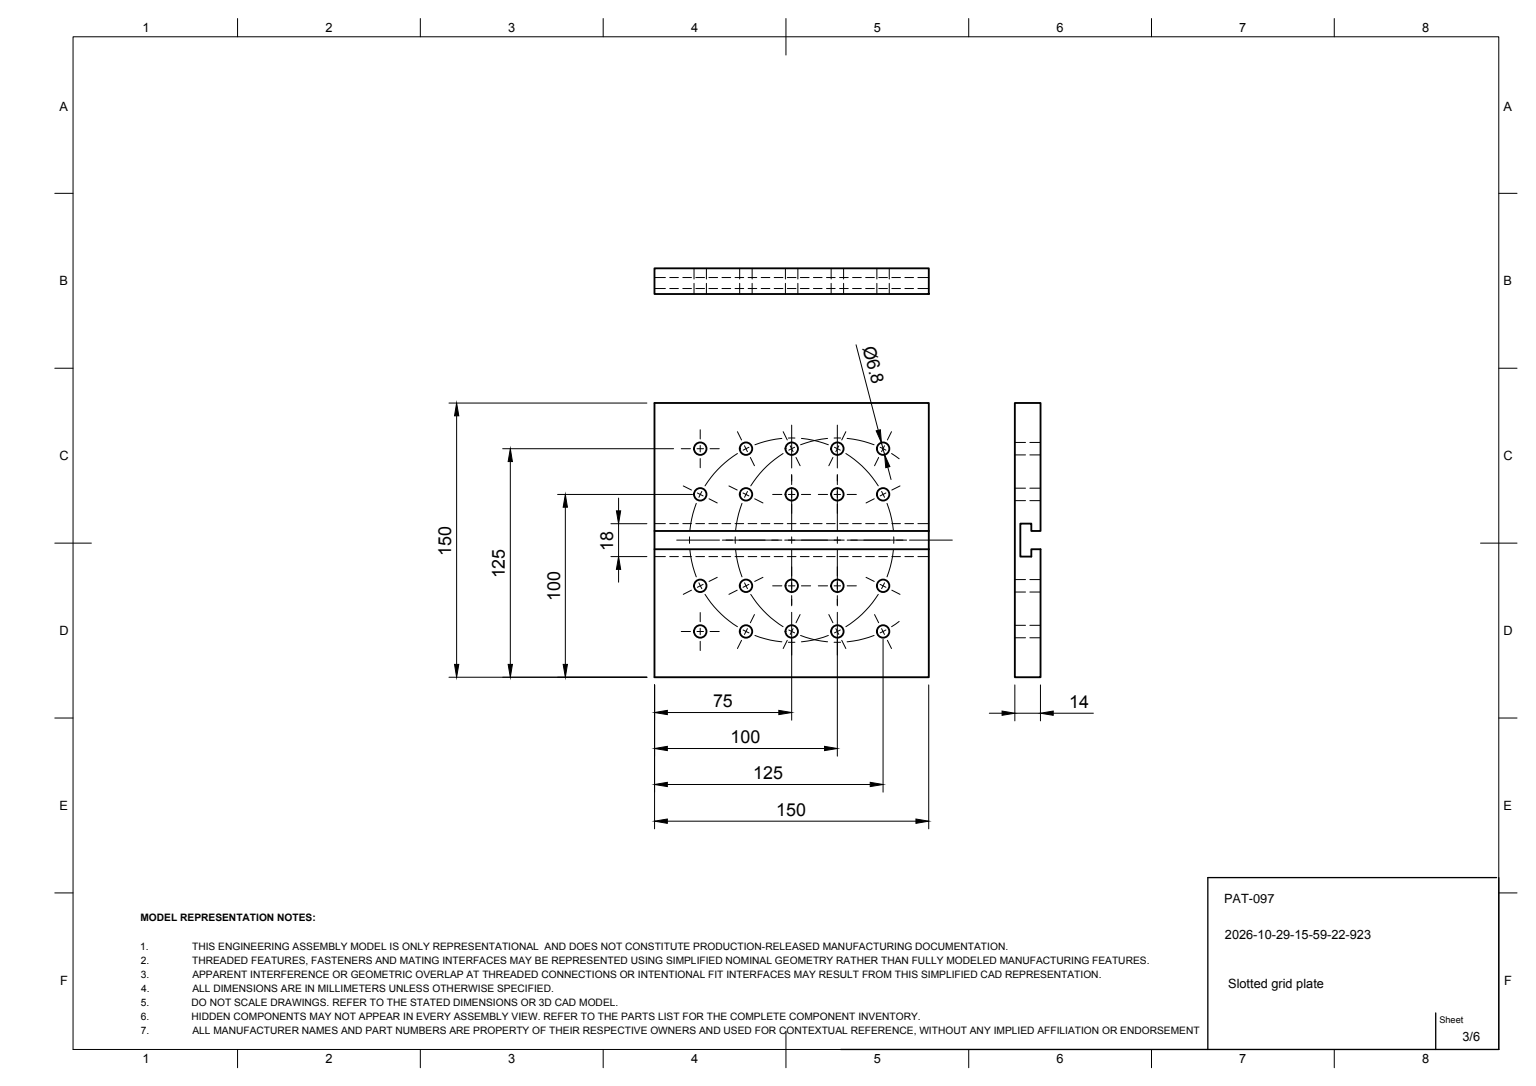
ISO-10303-21;
HEADER;
/* Generated by software containing ST-Developer
 * from STEP Tools, Inc. (www.steptools.com) 
 */

FILE_DESCRIPTION(
/* description */ ('PAT-097'),
/* implementation_level */ '2;1');

FILE_NAME(
/* name */ 'Slotted grid plate.step',
/* time_stamp */ '2026-10-29T15:59:31-07:00',
/* author */ (''),
/* organization */ (''),
/* preprocessor_version */ 'ST-DEVELOPER v20.2',
/* originating_system */ 'Autodesk Translation Framework v15.17.0.0',
/* authorisation */ '');

FILE_SCHEMA (('AUTOMOTIVE_DESIGN { 1 0 10303 214 3 1 1 }'));
ENDSEC;

DATA;
#10=MECHANICAL_DESIGN_GEOMETRIC_PRESENTATION_REPRESENTATION('',(#75),#2768);
#61=SHAPE_REPRESENTATION_RELATIONSHIP('SRR','None',#2799,#68);
#68=ADVANCED_BREP_SHAPE_REPRESENTATION('',(#82),#2761);
#75=STYLED_ITEM('',(#2925),#82);
#82=MANIFOLD_SOLID_BREP('Body1',#1596);
#89=CYLINDRICAL_SURFACE('',#1713,0.34);
#90=CYLINDRICAL_SURFACE('',#1715,0.34);
#91=CYLINDRICAL_SURFACE('',#1717,0.34);
#92=CYLINDRICAL_SURFACE('',#1719,0.34);
#93=CYLINDRICAL_SURFACE('',#1721,0.34);
#94=CYLINDRICAL_SURFACE('',#1723,0.34);
#95=CYLINDRICAL_SURFACE('',#1725,0.34);
#96=CYLINDRICAL_SURFACE('',#1727,0.34);
#97=CYLINDRICAL_SURFACE('',#1729,0.34);
#98=CYLINDRICAL_SURFACE('',#1731,0.34);
#99=CYLINDRICAL_SURFACE('',#1733,0.34);
#100=CYLINDRICAL_SURFACE('',#1735,0.34);
#101=CYLINDRICAL_SURFACE('',#1737,0.34);
#102=CYLINDRICAL_SURFACE('',#1739,0.34);
#103=CYLINDRICAL_SURFACE('',#1741,0.34);
#104=CYLINDRICAL_SURFACE('',#1743,0.34);
#105=CYLINDRICAL_SURFACE('',#1745,0.34);
#106=CYLINDRICAL_SURFACE('',#1747,0.34);
#107=CYLINDRICAL_SURFACE('',#1749,0.34);
#108=CYLINDRICAL_SURFACE('',#1751,0.34);
#116=FACE_BOUND('',#312,.T.);
#117=FACE_BOUND('',#313,.T.);
#118=FACE_BOUND('',#314,.T.);
#119=FACE_BOUND('',#315,.T.);
#120=FACE_BOUND('',#316,.T.);
#121=FACE_BOUND('',#317,.T.);
#122=FACE_BOUND('',#318,.T.);
#123=FACE_BOUND('',#319,.T.);
#124=FACE_BOUND('',#320,.T.);
#125=FACE_BOUND('',#321,.T.);
#126=FACE_BOUND('',#323,.T.);
#127=FACE_BOUND('',#324,.T.);
#128=FACE_BOUND('',#325,.T.);
#129=FACE_BOUND('',#326,.T.);
#130=FACE_BOUND('',#327,.T.);
#131=FACE_BOUND('',#328,.T.);
#132=FACE_BOUND('',#329,.T.);
#133=FACE_BOUND('',#330,.T.);
#134=FACE_BOUND('',#331,.T.);
#135=FACE_BOUND('',#332,.T.);
#136=FACE_BOUND('',#357,.T.);
#137=FACE_BOUND('',#358,.T.);
#138=FACE_BOUND('',#359,.T.);
#139=FACE_BOUND('',#360,.T.);
#140=FACE_BOUND('',#361,.T.);
#141=FACE_BOUND('',#362,.T.);
#142=FACE_BOUND('',#363,.T.);
#143=FACE_BOUND('',#364,.T.);
#144=FACE_BOUND('',#365,.T.);
#145=FACE_BOUND('',#366,.T.);
#146=FACE_BOUND('',#367,.T.);
#147=FACE_BOUND('',#368,.T.);
#148=FACE_BOUND('',#369,.T.);
#149=FACE_BOUND('',#370,.T.);
#150=FACE_BOUND('',#371,.T.);
#151=FACE_BOUND('',#372,.T.);
#152=FACE_BOUND('',#373,.T.);
#153=FACE_BOUND('',#374,.T.);
#154=FACE_BOUND('',#375,.T.);
#155=FACE_BOUND('',#376,.T.);
#164=CIRCLE('',#1692,0.34);
#165=CIRCLE('',#1693,0.34);
#166=CIRCLE('',#1694,0.34);
#167=CIRCLE('',#1695,0.34);
#168=CIRCLE('',#1696,0.34);
#169=CIRCLE('',#1697,0.34);
#170=CIRCLE('',#1698,0.34);
#171=CIRCLE('',#1699,0.34);
#172=CIRCLE('',#1700,0.34);
#173=CIRCLE('',#1701,0.34);
#174=CIRCLE('',#1703,0.34);
#175=CIRCLE('',#1704,0.34);
#176=CIRCLE('',#1705,0.34);
#177=CIRCLE('',#1706,0.34);
#178=CIRCLE('',#1707,0.34);
#179=CIRCLE('',#1708,0.34);
#180=CIRCLE('',#1709,0.34);
#181=CIRCLE('',#1710,0.34);
#182=CIRCLE('',#1711,0.34);
#183=CIRCLE('',#1712,0.34);
#184=CIRCLE('',#1714,0.34);
#185=CIRCLE('',#1716,0.34);
#186=CIRCLE('',#1718,0.34);
#187=CIRCLE('',#1720,0.34);
#188=CIRCLE('',#1722,0.34);
#189=CIRCLE('',#1724,0.34);
#190=CIRCLE('',#1726,0.34);
#191=CIRCLE('',#1728,0.34);
#192=CIRCLE('',#1730,0.34);
#193=CIRCLE('',#1732,0.34);
#194=CIRCLE('',#1734,0.34);
#195=CIRCLE('',#1736,0.34);
#196=CIRCLE('',#1738,0.34);
#197=CIRCLE('',#1740,0.34);
#198=CIRCLE('',#1742,0.34);
#199=CIRCLE('',#1744,0.34);
#200=CIRCLE('',#1746,0.34);
#201=CIRCLE('',#1748,0.34);
#202=CIRCLE('',#1750,0.34);
#203=CIRCLE('',#1752,0.34);
#220=FACE_OUTER_BOUND('',#303,.T.);
#221=FACE_OUTER_BOUND('',#304,.T.);
#222=FACE_OUTER_BOUND('',#305,.T.);
#223=FACE_OUTER_BOUND('',#306,.T.);
#224=FACE_OUTER_BOUND('',#307,.T.);
#225=FACE_OUTER_BOUND('',#308,.T.);
#226=FACE_OUTER_BOUND('',#309,.T.);
#227=FACE_OUTER_BOUND('',#310,.T.);
#228=FACE_OUTER_BOUND('',#311,.T.);
#229=FACE_OUTER_BOUND('',#322,.T.);
#230=FACE_OUTER_BOUND('',#333,.T.);
#231=FACE_OUTER_BOUND('',#334,.T.);
#232=FACE_OUTER_BOUND('',#335,.T.);
#233=FACE_OUTER_BOUND('',#336,.T.);
#234=FACE_OUTER_BOUND('',#337,.T.);
#235=FACE_OUTER_BOUND('',#338,.T.);
#236=FACE_OUTER_BOUND('',#339,.T.);
#237=FACE_OUTER_BOUND('',#340,.T.);
#238=FACE_OUTER_BOUND('',#341,.T.);
#239=FACE_OUTER_BOUND('',#342,.T.);
#240=FACE_OUTER_BOUND('',#343,.T.);
#241=FACE_OUTER_BOUND('',#344,.T.);
#242=FACE_OUTER_BOUND('',#345,.T.);
#243=FACE_OUTER_BOUND('',#346,.T.);
#244=FACE_OUTER_BOUND('',#347,.T.);
#245=FACE_OUTER_BOUND('',#348,.T.);
#246=FACE_OUTER_BOUND('',#349,.T.);
#247=FACE_OUTER_BOUND('',#350,.T.);
#248=FACE_OUTER_BOUND('',#351,.T.);
#249=FACE_OUTER_BOUND('',#352,.T.);
#250=FACE_OUTER_BOUND('',#353,.T.);
#251=FACE_OUTER_BOUND('',#354,.T.);
#252=FACE_OUTER_BOUND('',#355,.T.);
#253=FACE_OUTER_BOUND('',#356,.T.);
#303=EDGE_LOOP('',(#1049,#1050,#1051,#1052));
#304=EDGE_LOOP('',(#1053,#1054,#1055,#1056));
#305=EDGE_LOOP('',(#1057,#1058,#1059,#1060));
#306=EDGE_LOOP('',(#1061,#1062,#1063,#1064));
#307=EDGE_LOOP('',(#1065,#1066,#1067,#1068));
#308=EDGE_LOOP('',(#1069,#1070,#1071,#1072));
#309=EDGE_LOOP('',(#1073,#1074,#1075,#1076));
#310=EDGE_LOOP('',(#1077,#1078,#1079,#1080,#1081,#1082,#1083,#1084,#1085,
#1086,#1087,#1088));
#311=EDGE_LOOP('',(#1089,#1090,#1091,#1092));
#312=EDGE_LOOP('',(#1093));
#313=EDGE_LOOP('',(#1094));
#314=EDGE_LOOP('',(#1095));
#315=EDGE_LOOP('',(#1096));
#316=EDGE_LOOP('',(#1097));
#317=EDGE_LOOP('',(#1098));
#318=EDGE_LOOP('',(#1099));
#319=EDGE_LOOP('',(#1100));
#320=EDGE_LOOP('',(#1101));
#321=EDGE_LOOP('',(#1102));
#322=EDGE_LOOP('',(#1103,#1104,#1105,#1106));
#323=EDGE_LOOP('',(#1107));
#324=EDGE_LOOP('',(#1108));
#325=EDGE_LOOP('',(#1109));
#326=EDGE_LOOP('',(#1110));
#327=EDGE_LOOP('',(#1111));
#328=EDGE_LOOP('',(#1112));
#329=EDGE_LOOP('',(#1113));
#330=EDGE_LOOP('',(#1114));
#331=EDGE_LOOP('',(#1115));
#332=EDGE_LOOP('',(#1116));
#333=EDGE_LOOP('',(#1117,#1118,#1119,#1120));
#334=EDGE_LOOP('',(#1121,#1122,#1123,#1124));
#335=EDGE_LOOP('',(#1125,#1126,#1127,#1128));
#336=EDGE_LOOP('',(#1129,#1130,#1131,#1132));
#337=EDGE_LOOP('',(#1133,#1134,#1135,#1136));
#338=EDGE_LOOP('',(#1137,#1138,#1139,#1140));
#339=EDGE_LOOP('',(#1141,#1142,#1143,#1144));
#340=EDGE_LOOP('',(#1145,#1146,#1147,#1148));
#341=EDGE_LOOP('',(#1149,#1150,#1151,#1152));
#342=EDGE_LOOP('',(#1153,#1154,#1155,#1156));
#343=EDGE_LOOP('',(#1157,#1158,#1159,#1160));
#344=EDGE_LOOP('',(#1161,#1162,#1163,#1164));
#345=EDGE_LOOP('',(#1165,#1166,#1167,#1168));
#346=EDGE_LOOP('',(#1169,#1170,#1171,#1172));
#347=EDGE_LOOP('',(#1173,#1174,#1175,#1176));
#348=EDGE_LOOP('',(#1177,#1178,#1179,#1180));
#349=EDGE_LOOP('',(#1181,#1182,#1183,#1184));
#350=EDGE_LOOP('',(#1185,#1186,#1187,#1188));
#351=EDGE_LOOP('',(#1189,#1190,#1191,#1192));
#352=EDGE_LOOP('',(#1193,#1194,#1195,#1196));
#353=EDGE_LOOP('',(#1197,#1198,#1199,#1200));
#354=EDGE_LOOP('',(#1201,#1202,#1203,#1204,#1205,#1206,#1207,#1208,#1209,
#1210,#1211,#1212));
#355=EDGE_LOOP('',(#1213,#1214,#1215,#1216));
#356=EDGE_LOOP('',(#1217,#1218,#1219,#1220));
#357=EDGE_LOOP('',(#1221));
#358=EDGE_LOOP('',(#1222));
#359=EDGE_LOOP('',(#1223));
#360=EDGE_LOOP('',(#1224));
#361=EDGE_LOOP('',(#1225));
#362=EDGE_LOOP('',(#1226));
#363=EDGE_LOOP('',(#1227));
#364=EDGE_LOOP('',(#1228));
#365=EDGE_LOOP('',(#1229));
#366=EDGE_LOOP('',(#1230));
#367=EDGE_LOOP('',(#1231));
#368=EDGE_LOOP('',(#1232));
#369=EDGE_LOOP('',(#1233));
#370=EDGE_LOOP('',(#1234));
#371=EDGE_LOOP('',(#1235));
#372=EDGE_LOOP('',(#1236));
#373=EDGE_LOOP('',(#1237));
#374=EDGE_LOOP('',(#1238));
#375=EDGE_LOOP('',(#1239));
#376=EDGE_LOOP('',(#1240));
#434=LINE('',#2291,#571);
#435=LINE('',#2293,#572);
#436=LINE('',#2295,#573);
#437=LINE('',#2296,#574);
#438=LINE('',#2299,#575);
#439=LINE('',#2301,#576);
#440=LINE('',#2302,#577);
#441=LINE('',#2306,#578);
#442=LINE('',#2308,#579);
#443=LINE('',#2310,#580);
#444=LINE('',#2311,#581);
#445=LINE('',#2314,#582);
#446=LINE('',#2316,#583);
#447=LINE('',#2317,#584);
#448=LINE('',#2320,#585);
#449=LINE('',#2322,#586);
#450=LINE('',#2323,#587);
#451=LINE('',#2326,#588);
#452=LINE('',#2328,#589);
#453=LINE('',#2329,#590);
#454=LINE('',#2331,#591);
#455=LINE('',#2332,#592);
#456=LINE('',#2335,#593);
#457=LINE('',#2337,#594);
#458=LINE('',#2339,#595);
#459=LINE('',#2341,#596);
#460=LINE('',#2342,#597);
#461=LINE('',#2345,#598);
#462=LINE('',#2346,#599);
#463=LINE('',#2369,#600);
#464=LINE('',#2370,#601);
#465=LINE('',#2394,#602);
#466=LINE('',#2398,#603);
#467=LINE('',#2402,#604);
#468=LINE('',#2406,#605);
#469=LINE('',#2410,#606);
#470=LINE('',#2414,#607);
#471=LINE('',#2418,#608);
#472=LINE('',#2422,#609);
#473=LINE('',#2426,#610);
#474=LINE('',#2430,#611);
#475=LINE('',#2434,#612);
#476=LINE('',#2438,#613);
#477=LINE('',#2442,#614);
#478=LINE('',#2446,#615);
#479=LINE('',#2450,#616);
#480=LINE('',#2454,#617);
#481=LINE('',#2458,#618);
#482=LINE('',#2462,#619);
#483=LINE('',#2466,#620);
#484=LINE('',#2470,#621);
#485=LINE('',#2473,#622);
#486=LINE('',#2474,#623);
#487=LINE('',#2477,#624);
#488=LINE('',#2478,#625);
#489=LINE('',#2480,#626);
#571=VECTOR('',#1843,1.);
#572=VECTOR('',#1844,1.);
#573=VECTOR('',#1845,1.);
#574=VECTOR('',#1846,1.);
#575=VECTOR('',#1849,1.);
#576=VECTOR('',#1850,1.);
#577=VECTOR('',#1851,1.);
#578=VECTOR('',#1854,1.);
#579=VECTOR('',#1855,1.);
#580=VECTOR('',#1856,1.);
#581=VECTOR('',#1857,1.);
#582=VECTOR('',#1860,1.);
#583=VECTOR('',#1861,1.);
#584=VECTOR('',#1862,1.);
#585=VECTOR('',#1865,1.);
#586=VECTOR('',#1866,1.);
#587=VECTOR('',#1867,1.);
#588=VECTOR('',#1870,1.);
#589=VECTOR('',#1871,1.);
#590=VECTOR('',#1872,1.);
#591=VECTOR('',#1875,1.);
#592=VECTOR('',#1876,1.);
#593=VECTOR('',#1879,1.);
#594=VECTOR('',#1880,1.);
#595=VECTOR('',#1881,1.);
#596=VECTOR('',#1882,1.);
#597=VECTOR('',#1883,1.);
#598=VECTOR('',#1886,1.);
#599=VECTOR('',#1887,1.);
#600=VECTOR('',#1910,1.);
#601=VECTOR('',#1911,1.);
#602=VECTOR('',#1936,0.34);
#603=VECTOR('',#1941,0.34);
#604=VECTOR('',#1946,0.34);
#605=VECTOR('',#1951,0.34);
#606=VECTOR('',#1956,0.34);
#607=VECTOR('',#1961,0.34);
#608=VECTOR('',#1966,0.34);
#609=VECTOR('',#1971,0.34);
#610=VECTOR('',#1976,0.34);
#611=VECTOR('',#1981,0.34);
#612=VECTOR('',#1986,0.34);
#613=VECTOR('',#1991,0.34);
#614=VECTOR('',#1996,0.34);
#615=VECTOR('',#2001,0.34);
#616=VECTOR('',#2006,0.34);
#617=VECTOR('',#2011,0.34);
#618=VECTOR('',#2016,0.34);
#619=VECTOR('',#2021,0.34);
#620=VECTOR('',#2026,0.34);
#621=VECTOR('',#2031,0.34);
#622=VECTOR('',#2034,1.);
#623=VECTOR('',#2035,1.);
#624=VECTOR('',#2038,1.);
#625=VECTOR('',#2039,1.);
#626=VECTOR('',#2042,1.);
#708=VERTEX_POINT('',#2289);
#709=VERTEX_POINT('',#2290);
#710=VERTEX_POINT('',#2292);
#711=VERTEX_POINT('',#2294);
#712=VERTEX_POINT('',#2298);
#713=VERTEX_POINT('',#2300);
#714=VERTEX_POINT('',#2304);
#715=VERTEX_POINT('',#2305);
#716=VERTEX_POINT('',#2307);
#717=VERTEX_POINT('',#2309);
#718=VERTEX_POINT('',#2313);
#719=VERTEX_POINT('',#2315);
#720=VERTEX_POINT('',#2319);
#721=VERTEX_POINT('',#2321);
#722=VERTEX_POINT('',#2325);
#723=VERTEX_POINT('',#2327);
#724=VERTEX_POINT('',#2334);
#725=VERTEX_POINT('',#2336);
#726=VERTEX_POINT('',#2338);
#727=VERTEX_POINT('',#2340);
#728=VERTEX_POINT('',#2344);
#729=VERTEX_POINT('',#2347);
#730=VERTEX_POINT('',#2349);
#731=VERTEX_POINT('',#2351);
#732=VERTEX_POINT('',#2353);
#733=VERTEX_POINT('',#2355);
#734=VERTEX_POINT('',#2357);
#735=VERTEX_POINT('',#2359);
#736=VERTEX_POINT('',#2361);
#737=VERTEX_POINT('',#2363);
#738=VERTEX_POINT('',#2365);
#739=VERTEX_POINT('',#2368);
#740=VERTEX_POINT('',#2371);
#741=VERTEX_POINT('',#2373);
#742=VERTEX_POINT('',#2375);
#743=VERTEX_POINT('',#2377);
#744=VERTEX_POINT('',#2379);
#745=VERTEX_POINT('',#2381);
#746=VERTEX_POINT('',#2383);
#747=VERTEX_POINT('',#2385);
#748=VERTEX_POINT('',#2387);
#749=VERTEX_POINT('',#2389);
#750=VERTEX_POINT('',#2392);
#751=VERTEX_POINT('',#2396);
#752=VERTEX_POINT('',#2400);
#753=VERTEX_POINT('',#2404);
#754=VERTEX_POINT('',#2408);
#755=VERTEX_POINT('',#2412);
#756=VERTEX_POINT('',#2416);
#757=VERTEX_POINT('',#2420);
#758=VERTEX_POINT('',#2424);
#759=VERTEX_POINT('',#2428);
#760=VERTEX_POINT('',#2432);
#761=VERTEX_POINT('',#2436);
#762=VERTEX_POINT('',#2440);
#763=VERTEX_POINT('',#2444);
#764=VERTEX_POINT('',#2448);
#765=VERTEX_POINT('',#2452);
#766=VERTEX_POINT('',#2456);
#767=VERTEX_POINT('',#2460);
#768=VERTEX_POINT('',#2464);
#769=VERTEX_POINT('',#2468);
#770=VERTEX_POINT('',#2472);
#771=VERTEX_POINT('',#2476);
#844=EDGE_CURVE('',#708,#709,#434,.T.);
#845=EDGE_CURVE('',#710,#708,#435,.T.);
#846=EDGE_CURVE('',#711,#710,#436,.T.);
#847=EDGE_CURVE('',#709,#711,#437,.T.);
#848=EDGE_CURVE('',#712,#708,#438,.T.);
#849=EDGE_CURVE('',#713,#712,#439,.T.);
#850=EDGE_CURVE('',#710,#713,#440,.T.);
#851=EDGE_CURVE('',#714,#715,#441,.T.);
#852=EDGE_CURVE('',#716,#714,#442,.T.);
#853=EDGE_CURVE('',#717,#716,#443,.T.);
#854=EDGE_CURVE('',#717,#715,#444,.T.);
#855=EDGE_CURVE('',#715,#718,#445,.T.);
#856=EDGE_CURVE('',#719,#717,#446,.T.);
#857=EDGE_CURVE('',#719,#718,#447,.T.);
#858=EDGE_CURVE('',#718,#720,#448,.T.);
#859=EDGE_CURVE('',#721,#719,#449,.T.);
#860=EDGE_CURVE('',#721,#720,#450,.T.);
#861=EDGE_CURVE('',#720,#722,#451,.T.);
#862=EDGE_CURVE('',#723,#721,#452,.T.);
#863=EDGE_CURVE('',#723,#722,#453,.T.);
#864=EDGE_CURVE('',#722,#712,#454,.T.);
#865=EDGE_CURVE('',#713,#723,#455,.T.);
#866=EDGE_CURVE('',#724,#716,#456,.T.);
#867=EDGE_CURVE('',#725,#724,#457,.T.);
#868=EDGE_CURVE('',#725,#726,#458,.T.);
#869=EDGE_CURVE('',#726,#727,#459,.T.);
#870=EDGE_CURVE('',#711,#727,#460,.T.);
#871=EDGE_CURVE('',#714,#728,#461,.T.);
#872=EDGE_CURVE('',#728,#724,#462,.T.);
#873=EDGE_CURVE('',#729,#729,#164,.T.);
#874=EDGE_CURVE('',#730,#730,#165,.T.);
#875=EDGE_CURVE('',#731,#731,#166,.T.);
#876=EDGE_CURVE('',#732,#732,#167,.T.);
#877=EDGE_CURVE('',#733,#733,#168,.T.);
#878=EDGE_CURVE('',#734,#734,#169,.T.);
#879=EDGE_CURVE('',#735,#735,#170,.T.);
#880=EDGE_CURVE('',#736,#736,#171,.T.);
#881=EDGE_CURVE('',#737,#737,#172,.T.);
#882=EDGE_CURVE('',#738,#738,#173,.T.);
#883=EDGE_CURVE('',#727,#739,#463,.T.);
#884=EDGE_CURVE('',#739,#709,#464,.T.);
#885=EDGE_CURVE('',#740,#740,#174,.T.);
#886=EDGE_CURVE('',#741,#741,#175,.T.);
#887=EDGE_CURVE('',#742,#742,#176,.T.);
#888=EDGE_CURVE('',#743,#743,#177,.T.);
#889=EDGE_CURVE('',#744,#744,#178,.T.);
#890=EDGE_CURVE('',#745,#745,#179,.T.);
#891=EDGE_CURVE('',#746,#746,#180,.T.);
#892=EDGE_CURVE('',#747,#747,#181,.T.);
#893=EDGE_CURVE('',#748,#748,#182,.T.);
#894=EDGE_CURVE('',#749,#749,#183,.T.);
#895=EDGE_CURVE('',#750,#750,#184,.T.);
#896=EDGE_CURVE('',#750,#729,#465,.T.);
#897=EDGE_CURVE('',#751,#751,#185,.T.);
#898=EDGE_CURVE('',#751,#740,#466,.T.);
#899=EDGE_CURVE('',#752,#752,#186,.T.);
#900=EDGE_CURVE('',#752,#730,#467,.T.);
#901=EDGE_CURVE('',#753,#753,#187,.T.);
#902=EDGE_CURVE('',#753,#741,#468,.T.);
#903=EDGE_CURVE('',#754,#754,#188,.T.);
#904=EDGE_CURVE('',#754,#731,#469,.T.);
#905=EDGE_CURVE('',#755,#755,#189,.T.);
#906=EDGE_CURVE('',#755,#742,#470,.T.);
#907=EDGE_CURVE('',#756,#756,#190,.T.);
#908=EDGE_CURVE('',#756,#732,#471,.T.);
#909=EDGE_CURVE('',#757,#757,#191,.T.);
#910=EDGE_CURVE('',#757,#743,#472,.T.);
#911=EDGE_CURVE('',#758,#758,#192,.T.);
#912=EDGE_CURVE('',#758,#733,#473,.T.);
#913=EDGE_CURVE('',#759,#759,#193,.T.);
#914=EDGE_CURVE('',#759,#744,#474,.T.);
#915=EDGE_CURVE('',#760,#760,#194,.T.);
#916=EDGE_CURVE('',#760,#734,#475,.T.);
#917=EDGE_CURVE('',#761,#761,#195,.T.);
#918=EDGE_CURVE('',#761,#745,#476,.T.);
#919=EDGE_CURVE('',#762,#762,#196,.T.);
#920=EDGE_CURVE('',#762,#735,#477,.T.);
#921=EDGE_CURVE('',#763,#763,#197,.T.);
#922=EDGE_CURVE('',#763,#746,#478,.T.);
#923=EDGE_CURVE('',#764,#764,#198,.T.);
#924=EDGE_CURVE('',#764,#747,#479,.T.);
#925=EDGE_CURVE('',#765,#765,#199,.T.);
#926=EDGE_CURVE('',#765,#736,#480,.T.);
#927=EDGE_CURVE('',#766,#766,#200,.T.);
#928=EDGE_CURVE('',#766,#748,#481,.T.);
#929=EDGE_CURVE('',#767,#767,#201,.T.);
#930=EDGE_CURVE('',#767,#737,#482,.T.);
#931=EDGE_CURVE('',#768,#768,#202,.T.);
#932=EDGE_CURVE('',#768,#749,#483,.T.);
#933=EDGE_CURVE('',#769,#769,#203,.T.);
#934=EDGE_CURVE('',#769,#738,#484,.T.);
#935=EDGE_CURVE('',#770,#725,#485,.T.);
#936=EDGE_CURVE('',#770,#728,#486,.T.);
#937=EDGE_CURVE('',#771,#739,#487,.T.);
#938=EDGE_CURVE('',#771,#770,#488,.T.);
#939=EDGE_CURVE('',#726,#771,#489,.T.);
#1049=ORIENTED_EDGE('',*,*,#844,.F.);
#1050=ORIENTED_EDGE('',*,*,#845,.F.);
#1051=ORIENTED_EDGE('',*,*,#846,.F.);
#1052=ORIENTED_EDGE('',*,*,#847,.F.);
#1053=ORIENTED_EDGE('',*,*,#848,.F.);
#1054=ORIENTED_EDGE('',*,*,#849,.F.);
#1055=ORIENTED_EDGE('',*,*,#850,.F.);
#1056=ORIENTED_EDGE('',*,*,#845,.T.);
#1057=ORIENTED_EDGE('',*,*,#851,.F.);
#1058=ORIENTED_EDGE('',*,*,#852,.F.);
#1059=ORIENTED_EDGE('',*,*,#853,.F.);
#1060=ORIENTED_EDGE('',*,*,#854,.T.);
#1061=ORIENTED_EDGE('',*,*,#855,.F.);
#1062=ORIENTED_EDGE('',*,*,#854,.F.);
#1063=ORIENTED_EDGE('',*,*,#856,.F.);
#1064=ORIENTED_EDGE('',*,*,#857,.T.);
#1065=ORIENTED_EDGE('',*,*,#858,.F.);
#1066=ORIENTED_EDGE('',*,*,#857,.F.);
#1067=ORIENTED_EDGE('',*,*,#859,.F.);
#1068=ORIENTED_EDGE('',*,*,#860,.T.);
#1069=ORIENTED_EDGE('',*,*,#861,.F.);
#1070=ORIENTED_EDGE('',*,*,#860,.F.);
#1071=ORIENTED_EDGE('',*,*,#862,.F.);
#1072=ORIENTED_EDGE('',*,*,#863,.T.);
#1073=ORIENTED_EDGE('',*,*,#864,.F.);
#1074=ORIENTED_EDGE('',*,*,#863,.F.);
#1075=ORIENTED_EDGE('',*,*,#865,.F.);
#1076=ORIENTED_EDGE('',*,*,#849,.T.);
#1077=ORIENTED_EDGE('',*,*,#846,.T.);
#1078=ORIENTED_EDGE('',*,*,#850,.T.);
#1079=ORIENTED_EDGE('',*,*,#865,.T.);
#1080=ORIENTED_EDGE('',*,*,#862,.T.);
#1081=ORIENTED_EDGE('',*,*,#859,.T.);
#1082=ORIENTED_EDGE('',*,*,#856,.T.);
#1083=ORIENTED_EDGE('',*,*,#853,.T.);
#1084=ORIENTED_EDGE('',*,*,#866,.F.);
#1085=ORIENTED_EDGE('',*,*,#867,.F.);
#1086=ORIENTED_EDGE('',*,*,#868,.T.);
#1087=ORIENTED_EDGE('',*,*,#869,.T.);
#1088=ORIENTED_EDGE('',*,*,#870,.F.);
#1089=ORIENTED_EDGE('',*,*,#852,.T.);
#1090=ORIENTED_EDGE('',*,*,#871,.T.);
#1091=ORIENTED_EDGE('',*,*,#872,.T.);
#1092=ORIENTED_EDGE('',*,*,#866,.T.);
#1093=ORIENTED_EDGE('',*,*,#873,.T.);
#1094=ORIENTED_EDGE('',*,*,#874,.T.);
#1095=ORIENTED_EDGE('',*,*,#875,.T.);
#1096=ORIENTED_EDGE('',*,*,#876,.T.);
#1097=ORIENTED_EDGE('',*,*,#877,.T.);
#1098=ORIENTED_EDGE('',*,*,#878,.T.);
#1099=ORIENTED_EDGE('',*,*,#879,.T.);
#1100=ORIENTED_EDGE('',*,*,#880,.T.);
#1101=ORIENTED_EDGE('',*,*,#881,.T.);
#1102=ORIENTED_EDGE('',*,*,#882,.T.);
#1103=ORIENTED_EDGE('',*,*,#847,.T.);
#1104=ORIENTED_EDGE('',*,*,#870,.T.);
#1105=ORIENTED_EDGE('',*,*,#883,.T.);
#1106=ORIENTED_EDGE('',*,*,#884,.T.);
#1107=ORIENTED_EDGE('',*,*,#885,.T.);
#1108=ORIENTED_EDGE('',*,*,#886,.T.);
#1109=ORIENTED_EDGE('',*,*,#887,.T.);
#1110=ORIENTED_EDGE('',*,*,#888,.T.);
#1111=ORIENTED_EDGE('',*,*,#889,.T.);
#1112=ORIENTED_EDGE('',*,*,#890,.T.);
#1113=ORIENTED_EDGE('',*,*,#891,.T.);
#1114=ORIENTED_EDGE('',*,*,#892,.T.);
#1115=ORIENTED_EDGE('',*,*,#893,.T.);
#1116=ORIENTED_EDGE('',*,*,#894,.T.);
#1117=ORIENTED_EDGE('',*,*,#895,.F.);
#1118=ORIENTED_EDGE('',*,*,#896,.T.);
#1119=ORIENTED_EDGE('',*,*,#873,.F.);
#1120=ORIENTED_EDGE('',*,*,#896,.F.);
#1121=ORIENTED_EDGE('',*,*,#897,.F.);
#1122=ORIENTED_EDGE('',*,*,#898,.T.);
#1123=ORIENTED_EDGE('',*,*,#885,.F.);
#1124=ORIENTED_EDGE('',*,*,#898,.F.);
#1125=ORIENTED_EDGE('',*,*,#899,.F.);
#1126=ORIENTED_EDGE('',*,*,#900,.T.);
#1127=ORIENTED_EDGE('',*,*,#874,.F.);
#1128=ORIENTED_EDGE('',*,*,#900,.F.);
#1129=ORIENTED_EDGE('',*,*,#901,.F.);
#1130=ORIENTED_EDGE('',*,*,#902,.T.);
#1131=ORIENTED_EDGE('',*,*,#886,.F.);
#1132=ORIENTED_EDGE('',*,*,#902,.F.);
#1133=ORIENTED_EDGE('',*,*,#903,.F.);
#1134=ORIENTED_EDGE('',*,*,#904,.T.);
#1135=ORIENTED_EDGE('',*,*,#875,.F.);
#1136=ORIENTED_EDGE('',*,*,#904,.F.);
#1137=ORIENTED_EDGE('',*,*,#905,.F.);
#1138=ORIENTED_EDGE('',*,*,#906,.T.);
#1139=ORIENTED_EDGE('',*,*,#887,.F.);
#1140=ORIENTED_EDGE('',*,*,#906,.F.);
#1141=ORIENTED_EDGE('',*,*,#907,.F.);
#1142=ORIENTED_EDGE('',*,*,#908,.T.);
#1143=ORIENTED_EDGE('',*,*,#876,.F.);
#1144=ORIENTED_EDGE('',*,*,#908,.F.);
#1145=ORIENTED_EDGE('',*,*,#909,.F.);
#1146=ORIENTED_EDGE('',*,*,#910,.T.);
#1147=ORIENTED_EDGE('',*,*,#888,.F.);
#1148=ORIENTED_EDGE('',*,*,#910,.F.);
#1149=ORIENTED_EDGE('',*,*,#911,.F.);
#1150=ORIENTED_EDGE('',*,*,#912,.T.);
#1151=ORIENTED_EDGE('',*,*,#877,.F.);
#1152=ORIENTED_EDGE('',*,*,#912,.F.);
#1153=ORIENTED_EDGE('',*,*,#913,.F.);
#1154=ORIENTED_EDGE('',*,*,#914,.T.);
#1155=ORIENTED_EDGE('',*,*,#889,.F.);
#1156=ORIENTED_EDGE('',*,*,#914,.F.);
#1157=ORIENTED_EDGE('',*,*,#915,.F.);
#1158=ORIENTED_EDGE('',*,*,#916,.T.);
#1159=ORIENTED_EDGE('',*,*,#878,.F.);
#1160=ORIENTED_EDGE('',*,*,#916,.F.);
#1161=ORIENTED_EDGE('',*,*,#917,.F.);
#1162=ORIENTED_EDGE('',*,*,#918,.T.);
#1163=ORIENTED_EDGE('',*,*,#890,.F.);
#1164=ORIENTED_EDGE('',*,*,#918,.F.);
#1165=ORIENTED_EDGE('',*,*,#919,.F.);
#1166=ORIENTED_EDGE('',*,*,#920,.T.);
#1167=ORIENTED_EDGE('',*,*,#879,.F.);
#1168=ORIENTED_EDGE('',*,*,#920,.F.);
#1169=ORIENTED_EDGE('',*,*,#921,.F.);
#1170=ORIENTED_EDGE('',*,*,#922,.T.);
#1171=ORIENTED_EDGE('',*,*,#891,.F.);
#1172=ORIENTED_EDGE('',*,*,#922,.F.);
#1173=ORIENTED_EDGE('',*,*,#923,.F.);
#1174=ORIENTED_EDGE('',*,*,#924,.T.);
#1175=ORIENTED_EDGE('',*,*,#892,.F.);
#1176=ORIENTED_EDGE('',*,*,#924,.F.);
#1177=ORIENTED_EDGE('',*,*,#925,.F.);
#1178=ORIENTED_EDGE('',*,*,#926,.T.);
#1179=ORIENTED_EDGE('',*,*,#880,.F.);
#1180=ORIENTED_EDGE('',*,*,#926,.F.);
#1181=ORIENTED_EDGE('',*,*,#927,.F.);
#1182=ORIENTED_EDGE('',*,*,#928,.T.);
#1183=ORIENTED_EDGE('',*,*,#893,.F.);
#1184=ORIENTED_EDGE('',*,*,#928,.F.);
#1185=ORIENTED_EDGE('',*,*,#929,.F.);
#1186=ORIENTED_EDGE('',*,*,#930,.T.);
#1187=ORIENTED_EDGE('',*,*,#881,.F.);
#1188=ORIENTED_EDGE('',*,*,#930,.F.);
#1189=ORIENTED_EDGE('',*,*,#931,.F.);
#1190=ORIENTED_EDGE('',*,*,#932,.T.);
#1191=ORIENTED_EDGE('',*,*,#894,.F.);
#1192=ORIENTED_EDGE('',*,*,#932,.F.);
#1193=ORIENTED_EDGE('',*,*,#933,.F.);
#1194=ORIENTED_EDGE('',*,*,#934,.T.);
#1195=ORIENTED_EDGE('',*,*,#882,.F.);
#1196=ORIENTED_EDGE('',*,*,#934,.F.);
#1197=ORIENTED_EDGE('',*,*,#935,.T.);
#1198=ORIENTED_EDGE('',*,*,#867,.T.);
#1199=ORIENTED_EDGE('',*,*,#872,.F.);
#1200=ORIENTED_EDGE('',*,*,#936,.F.);
#1201=ORIENTED_EDGE('',*,*,#844,.T.);
#1202=ORIENTED_EDGE('',*,*,#884,.F.);
#1203=ORIENTED_EDGE('',*,*,#937,.F.);
#1204=ORIENTED_EDGE('',*,*,#938,.T.);
#1205=ORIENTED_EDGE('',*,*,#936,.T.);
#1206=ORIENTED_EDGE('',*,*,#871,.F.);
#1207=ORIENTED_EDGE('',*,*,#851,.T.);
#1208=ORIENTED_EDGE('',*,*,#855,.T.);
#1209=ORIENTED_EDGE('',*,*,#858,.T.);
#1210=ORIENTED_EDGE('',*,*,#861,.T.);
#1211=ORIENTED_EDGE('',*,*,#864,.T.);
#1212=ORIENTED_EDGE('',*,*,#848,.T.);
#1213=ORIENTED_EDGE('',*,*,#939,.T.);
#1214=ORIENTED_EDGE('',*,*,#937,.T.);
#1215=ORIENTED_EDGE('',*,*,#883,.F.);
#1216=ORIENTED_EDGE('',*,*,#869,.F.);
#1217=ORIENTED_EDGE('',*,*,#868,.F.);
#1218=ORIENTED_EDGE('',*,*,#935,.F.);
#1219=ORIENTED_EDGE('',*,*,#938,.F.);
#1220=ORIENTED_EDGE('',*,*,#939,.F.);
#1221=ORIENTED_EDGE('',*,*,#933,.T.);
#1222=ORIENTED_EDGE('',*,*,#931,.T.);
#1223=ORIENTED_EDGE('',*,*,#929,.T.);
#1224=ORIENTED_EDGE('',*,*,#927,.T.);
#1225=ORIENTED_EDGE('',*,*,#925,.T.);
#1226=ORIENTED_EDGE('',*,*,#923,.T.);
#1227=ORIENTED_EDGE('',*,*,#921,.T.);
#1228=ORIENTED_EDGE('',*,*,#919,.T.);
#1229=ORIENTED_EDGE('',*,*,#917,.T.);
#1230=ORIENTED_EDGE('',*,*,#915,.T.);
#1231=ORIENTED_EDGE('',*,*,#913,.T.);
#1232=ORIENTED_EDGE('',*,*,#911,.T.);
#1233=ORIENTED_EDGE('',*,*,#909,.T.);
#1234=ORIENTED_EDGE('',*,*,#907,.T.);
#1235=ORIENTED_EDGE('',*,*,#905,.T.);
#1236=ORIENTED_EDGE('',*,*,#903,.T.);
#1237=ORIENTED_EDGE('',*,*,#901,.T.);
#1238=ORIENTED_EDGE('',*,*,#899,.T.);
#1239=ORIENTED_EDGE('',*,*,#897,.T.);
#1240=ORIENTED_EDGE('',*,*,#895,.T.);
#1459=PLANE('',#1683);
#1460=PLANE('',#1684);
#1461=PLANE('',#1685);
#1462=PLANE('',#1686);
#1463=PLANE('',#1687);
#1464=PLANE('',#1688);
#1465=PLANE('',#1689);
#1466=PLANE('',#1690);
#1467=PLANE('',#1691);
#1468=PLANE('',#1702);
#1469=PLANE('',#1753);
#1470=PLANE('',#1754);
#1471=PLANE('',#1755);
#1472=PLANE('',#1756);
#1513=ADVANCED_FACE('',(#220),#1459,.F.);
#1514=ADVANCED_FACE('',(#221),#1460,.F.);
#1515=ADVANCED_FACE('',(#222),#1461,.F.);
#1516=ADVANCED_FACE('',(#223),#1462,.F.);
#1517=ADVANCED_FACE('',(#224),#1463,.F.);
#1518=ADVANCED_FACE('',(#225),#1464,.F.);
#1519=ADVANCED_FACE('',(#226),#1465,.F.);
#1520=ADVANCED_FACE('',(#227),#1466,.T.);
#1521=ADVANCED_FACE('',(#228,#116,#117,#118,#119,#120,#121,#122,#123,#124,
#125),#1467,.T.);
#1522=ADVANCED_FACE('',(#229,#126,#127,#128,#129,#130,#131,#132,#133,#134,
#135),#1468,.T.);
#1523=ADVANCED_FACE('',(#230),#89,.F.);
#1524=ADVANCED_FACE('',(#231),#90,.F.);
#1525=ADVANCED_FACE('',(#232),#91,.F.);
#1526=ADVANCED_FACE('',(#233),#92,.F.);
#1527=ADVANCED_FACE('',(#234),#93,.F.);
#1528=ADVANCED_FACE('',(#235),#94,.F.);
#1529=ADVANCED_FACE('',(#236),#95,.F.);
#1530=ADVANCED_FACE('',(#237),#96,.F.);
#1531=ADVANCED_FACE('',(#238),#97,.F.);
#1532=ADVANCED_FACE('',(#239),#98,.F.);
#1533=ADVANCED_FACE('',(#240),#99,.F.);
#1534=ADVANCED_FACE('',(#241),#100,.F.);
#1535=ADVANCED_FACE('',(#242),#101,.F.);
#1536=ADVANCED_FACE('',(#243),#102,.F.);
#1537=ADVANCED_FACE('',(#244),#103,.F.);
#1538=ADVANCED_FACE('',(#245),#104,.F.);
#1539=ADVANCED_FACE('',(#246),#105,.F.);
#1540=ADVANCED_FACE('',(#247),#106,.F.);
#1541=ADVANCED_FACE('',(#248),#107,.F.);
#1542=ADVANCED_FACE('',(#249),#108,.F.);
#1543=ADVANCED_FACE('',(#250),#1469,.T.);
#1544=ADVANCED_FACE('',(#251),#1470,.T.);
#1545=ADVANCED_FACE('',(#252),#1471,.T.);
#1546=ADVANCED_FACE('',(#253,#136,#137,#138,#139,#140,#141,#142,#143,#144,
#145,#146,#147,#148,#149,#150,#151,#152,#153,#154,#155),#1472,.F.);
#1596=CLOSED_SHELL('',(#1513,#1514,#1515,#1516,#1517,#1518,#1519,#1520,
#1521,#1522,#1523,#1524,#1525,#1526,#1527,#1528,#1529,#1530,#1531,#1532,
#1533,#1534,#1535,#1536,#1537,#1538,#1539,#1540,#1541,#1542,#1543,#1544,
#1545,#1546));
#1682=AXIS2_PLACEMENT_3D('',#2287,#1839,#1840);
#1683=AXIS2_PLACEMENT_3D('',#2288,#1841,#1842);
#1684=AXIS2_PLACEMENT_3D('',#2297,#1847,#1848);
#1685=AXIS2_PLACEMENT_3D('',#2303,#1852,#1853);
#1686=AXIS2_PLACEMENT_3D('',#2312,#1858,#1859);
#1687=AXIS2_PLACEMENT_3D('',#2318,#1863,#1864);
#1688=AXIS2_PLACEMENT_3D('',#2324,#1868,#1869);
#1689=AXIS2_PLACEMENT_3D('',#2330,#1873,#1874);
#1690=AXIS2_PLACEMENT_3D('',#2333,#1877,#1878);
#1691=AXIS2_PLACEMENT_3D('',#2343,#1884,#1885);
#1692=AXIS2_PLACEMENT_3D('',#2348,#1888,#1889);
#1693=AXIS2_PLACEMENT_3D('',#2350,#1890,#1891);
#1694=AXIS2_PLACEMENT_3D('',#2352,#1892,#1893);
#1695=AXIS2_PLACEMENT_3D('',#2354,#1894,#1895);
#1696=AXIS2_PLACEMENT_3D('',#2356,#1896,#1897);
#1697=AXIS2_PLACEMENT_3D('',#2358,#1898,#1899);
#1698=AXIS2_PLACEMENT_3D('',#2360,#1900,#1901);
#1699=AXIS2_PLACEMENT_3D('',#2362,#1902,#1903);
#1700=AXIS2_PLACEMENT_3D('',#2364,#1904,#1905);
#1701=AXIS2_PLACEMENT_3D('',#2366,#1906,#1907);
#1702=AXIS2_PLACEMENT_3D('',#2367,#1908,#1909);
#1703=AXIS2_PLACEMENT_3D('',#2372,#1912,#1913);
#1704=AXIS2_PLACEMENT_3D('',#2374,#1914,#1915);
#1705=AXIS2_PLACEMENT_3D('',#2376,#1916,#1917);
#1706=AXIS2_PLACEMENT_3D('',#2378,#1918,#1919);
#1707=AXIS2_PLACEMENT_3D('',#2380,#1920,#1921);
#1708=AXIS2_PLACEMENT_3D('',#2382,#1922,#1923);
#1709=AXIS2_PLACEMENT_3D('',#2384,#1924,#1925);
#1710=AXIS2_PLACEMENT_3D('',#2386,#1926,#1927);
#1711=AXIS2_PLACEMENT_3D('',#2388,#1928,#1929);
#1712=AXIS2_PLACEMENT_3D('',#2390,#1930,#1931);
#1713=AXIS2_PLACEMENT_3D('',#2391,#1932,#1933);
#1714=AXIS2_PLACEMENT_3D('',#2393,#1934,#1935);
#1715=AXIS2_PLACEMENT_3D('',#2395,#1937,#1938);
#1716=AXIS2_PLACEMENT_3D('',#2397,#1939,#1940);
#1717=AXIS2_PLACEMENT_3D('',#2399,#1942,#1943);
#1718=AXIS2_PLACEMENT_3D('',#2401,#1944,#1945);
#1719=AXIS2_PLACEMENT_3D('',#2403,#1947,#1948);
#1720=AXIS2_PLACEMENT_3D('',#2405,#1949,#1950);
#1721=AXIS2_PLACEMENT_3D('',#2407,#1952,#1953);
#1722=AXIS2_PLACEMENT_3D('',#2409,#1954,#1955);
#1723=AXIS2_PLACEMENT_3D('',#2411,#1957,#1958);
#1724=AXIS2_PLACEMENT_3D('',#2413,#1959,#1960);
#1725=AXIS2_PLACEMENT_3D('',#2415,#1962,#1963);
#1726=AXIS2_PLACEMENT_3D('',#2417,#1964,#1965);
#1727=AXIS2_PLACEMENT_3D('',#2419,#1967,#1968);
#1728=AXIS2_PLACEMENT_3D('',#2421,#1969,#1970);
#1729=AXIS2_PLACEMENT_3D('',#2423,#1972,#1973);
#1730=AXIS2_PLACEMENT_3D('',#2425,#1974,#1975);
#1731=AXIS2_PLACEMENT_3D('',#2427,#1977,#1978);
#1732=AXIS2_PLACEMENT_3D('',#2429,#1979,#1980);
#1733=AXIS2_PLACEMENT_3D('',#2431,#1982,#1983);
#1734=AXIS2_PLACEMENT_3D('',#2433,#1984,#1985);
#1735=AXIS2_PLACEMENT_3D('',#2435,#1987,#1988);
#1736=AXIS2_PLACEMENT_3D('',#2437,#1989,#1990);
#1737=AXIS2_PLACEMENT_3D('',#2439,#1992,#1993);
#1738=AXIS2_PLACEMENT_3D('',#2441,#1994,#1995);
#1739=AXIS2_PLACEMENT_3D('',#2443,#1997,#1998);
#1740=AXIS2_PLACEMENT_3D('',#2445,#1999,#2000);
#1741=AXIS2_PLACEMENT_3D('',#2447,#2002,#2003);
#1742=AXIS2_PLACEMENT_3D('',#2449,#2004,#2005);
#1743=AXIS2_PLACEMENT_3D('',#2451,#2007,#2008);
#1744=AXIS2_PLACEMENT_3D('',#2453,#2009,#2010);
#1745=AXIS2_PLACEMENT_3D('',#2455,#2012,#2013);
#1746=AXIS2_PLACEMENT_3D('',#2457,#2014,#2015);
#1747=AXIS2_PLACEMENT_3D('',#2459,#2017,#2018);
#1748=AXIS2_PLACEMENT_3D('',#2461,#2019,#2020);
#1749=AXIS2_PLACEMENT_3D('',#2463,#2022,#2023);
#1750=AXIS2_PLACEMENT_3D('',#2465,#2024,#2025);
#1751=AXIS2_PLACEMENT_3D('',#2467,#2027,#2028);
#1752=AXIS2_PLACEMENT_3D('',#2469,#2029,#2030);
#1753=AXIS2_PLACEMENT_3D('',#2471,#2032,#2033);
#1754=AXIS2_PLACEMENT_3D('',#2475,#2036,#2037);
#1755=AXIS2_PLACEMENT_3D('',#2479,#2040,#2041);
#1756=AXIS2_PLACEMENT_3D('',#2481,#2043,#2044);
#1839=DIRECTION('axis',(0.,0.,1.));
#1840=DIRECTION('refdir',(1.,0.,0.));
#1841=DIRECTION('center_axis',(0.,-1.,0.));
#1842=DIRECTION('ref_axis',(0.,0.,-1.));
#1843=DIRECTION('',(0.,0.,1.));
#1844=DIRECTION('',(1.,0.,0.));
#1845=DIRECTION('',(0.,0.,-1.));
#1846=DIRECTION('',(-1.,0.,0.));
#1847=DIRECTION('center_axis',(0.,0.,1.));
#1848=DIRECTION('ref_axis',(0.,-1.,0.));
#1849=DIRECTION('',(0.,1.,0.));
#1850=DIRECTION('',(1.,0.,0.));
#1851=DIRECTION('',(0.,-1.,0.));
#1852=DIRECTION('center_axis',(0.,1.,0.));
#1853=DIRECTION('ref_axis',(0.,0.,1.));
#1854=DIRECTION('',(0.,0.,-1.));
#1855=DIRECTION('',(1.,0.,0.));
#1856=DIRECTION('',(0.,0.,1.));
#1857=DIRECTION('',(1.,0.,0.));
#1858=DIRECTION('center_axis',(0.,0.,1.));
#1859=DIRECTION('ref_axis',(0.,-1.,0.));
#1860=DIRECTION('',(0.,1.,0.));
#1861=DIRECTION('',(0.,-1.,0.));
#1862=DIRECTION('',(1.,0.,0.));
#1863=DIRECTION('center_axis',(0.,1.,0.));
#1864=DIRECTION('ref_axis',(0.,0.,1.));
#1865=DIRECTION('',(0.,0.,-1.));
#1866=DIRECTION('',(0.,0.,1.));
#1867=DIRECTION('',(1.,0.,0.));
#1868=DIRECTION('center_axis',(0.,0.,-1.));
#1869=DIRECTION('ref_axis',(0.,1.,0.));
#1870=DIRECTION('',(0.,-1.,0.));
#1871=DIRECTION('',(0.,1.,0.));
#1872=DIRECTION('',(1.,0.,0.));
#1873=DIRECTION('center_axis',(0.,-1.,0.));
#1874=DIRECTION('ref_axis',(0.,0.,-1.));
#1875=DIRECTION('',(0.,0.,1.));
#1876=DIRECTION('',(0.,0.,-1.));
#1877=DIRECTION('center_axis',(-1.,0.,0.));
#1878=DIRECTION('ref_axis',(0.,-1.,0.));
#1879=DIRECTION('',(0.,-1.,0.));
#1880=DIRECTION('',(0.,0.,1.));
#1881=DIRECTION('',(0.,-1.,0.));
#1882=DIRECTION('',(0.,0.,1.));
#1883=DIRECTION('',(0.,-1.,0.));
#1884=DIRECTION('center_axis',(0.,0.,1.));
#1885=DIRECTION('ref_axis',(1.,0.,0.));
#1886=DIRECTION('',(0.,1.,0.));
#1887=DIRECTION('',(-1.,0.,0.));
#1888=DIRECTION('center_axis',(0.,0.,-1.));
#1889=DIRECTION('ref_axis',(1.,0.,0.));
#1890=DIRECTION('center_axis',(0.,0.,-1.));
#1891=DIRECTION('ref_axis',(1.,0.,0.));
#1892=DIRECTION('center_axis',(0.,0.,-1.));
#1893=DIRECTION('ref_axis',(1.,0.,0.));
#1894=DIRECTION('center_axis',(0.,0.,-1.));
#1895=DIRECTION('ref_axis',(1.,0.,0.));
#1896=DIRECTION('center_axis',(0.,0.,-1.));
#1897=DIRECTION('ref_axis',(1.,0.,0.));
#1898=DIRECTION('center_axis',(0.,0.,-1.));
#1899=DIRECTION('ref_axis',(1.,0.,0.));
#1900=DIRECTION('center_axis',(0.,0.,-1.));
#1901=DIRECTION('ref_axis',(1.,0.,0.));
#1902=DIRECTION('center_axis',(0.,0.,-1.));
#1903=DIRECTION('ref_axis',(1.,0.,0.));
#1904=DIRECTION('center_axis',(0.,0.,-1.));
#1905=DIRECTION('ref_axis',(1.,0.,0.));
#1906=DIRECTION('center_axis',(0.,0.,-1.));
#1907=DIRECTION('ref_axis',(1.,0.,0.));
#1908=DIRECTION('center_axis',(0.,0.,1.));
#1909=DIRECTION('ref_axis',(1.,0.,0.));
#1910=DIRECTION('',(1.,0.,0.));
#1911=DIRECTION('',(0.,1.,0.));
#1912=DIRECTION('center_axis',(0.,0.,-1.));
#1913=DIRECTION('ref_axis',(1.,0.,0.));
#1914=DIRECTION('center_axis',(0.,0.,-1.));
#1915=DIRECTION('ref_axis',(1.,0.,0.));
#1916=DIRECTION('center_axis',(0.,0.,-1.));
#1917=DIRECTION('ref_axis',(1.,0.,0.));
#1918=DIRECTION('center_axis',(0.,0.,-1.));
#1919=DIRECTION('ref_axis',(1.,0.,0.));
#1920=DIRECTION('center_axis',(0.,0.,-1.));
#1921=DIRECTION('ref_axis',(1.,0.,0.));
#1922=DIRECTION('center_axis',(0.,0.,-1.));
#1923=DIRECTION('ref_axis',(1.,0.,0.));
#1924=DIRECTION('center_axis',(0.,0.,-1.));
#1925=DIRECTION('ref_axis',(1.,0.,0.));
#1926=DIRECTION('center_axis',(0.,0.,-1.));
#1927=DIRECTION('ref_axis',(1.,0.,0.));
#1928=DIRECTION('center_axis',(0.,0.,-1.));
#1929=DIRECTION('ref_axis',(1.,0.,0.));
#1930=DIRECTION('center_axis',(0.,0.,-1.));
#1931=DIRECTION('ref_axis',(1.,0.,0.));
#1932=DIRECTION('center_axis',(0.,0.,1.));
#1933=DIRECTION('ref_axis',(1.,0.,0.));
#1934=DIRECTION('center_axis',(0.,0.,1.));
#1935=DIRECTION('ref_axis',(1.,0.,0.));
#1936=DIRECTION('',(0.,0.,1.));
#1937=DIRECTION('center_axis',(0.,0.,1.));
#1938=DIRECTION('ref_axis',(1.,0.,0.));
#1939=DIRECTION('center_axis',(0.,0.,1.));
#1940=DIRECTION('ref_axis',(1.,0.,0.));
#1941=DIRECTION('',(0.,0.,1.));
#1942=DIRECTION('center_axis',(0.,0.,1.));
#1943=DIRECTION('ref_axis',(1.,0.,0.));
#1944=DIRECTION('center_axis',(0.,0.,1.));
#1945=DIRECTION('ref_axis',(1.,0.,0.));
#1946=DIRECTION('',(0.,0.,1.));
#1947=DIRECTION('center_axis',(0.,0.,1.));
#1948=DIRECTION('ref_axis',(1.,0.,0.));
#1949=DIRECTION('center_axis',(0.,0.,1.));
#1950=DIRECTION('ref_axis',(1.,0.,0.));
#1951=DIRECTION('',(0.,0.,1.));
#1952=DIRECTION('center_axis',(0.,0.,1.));
#1953=DIRECTION('ref_axis',(1.,0.,0.));
#1954=DIRECTION('center_axis',(0.,0.,1.));
#1955=DIRECTION('ref_axis',(1.,0.,0.));
#1956=DIRECTION('',(0.,0.,1.));
#1957=DIRECTION('center_axis',(0.,0.,1.));
#1958=DIRECTION('ref_axis',(1.,0.,0.));
#1959=DIRECTION('center_axis',(0.,0.,1.));
#1960=DIRECTION('ref_axis',(1.,0.,0.));
#1961=DIRECTION('',(0.,0.,1.));
#1962=DIRECTION('center_axis',(0.,0.,1.));
#1963=DIRECTION('ref_axis',(1.,0.,0.));
#1964=DIRECTION('center_axis',(0.,0.,1.));
#1965=DIRECTION('ref_axis',(1.,0.,0.));
#1966=DIRECTION('',(0.,0.,1.));
#1967=DIRECTION('center_axis',(0.,0.,1.));
#1968=DIRECTION('ref_axis',(1.,0.,0.));
#1969=DIRECTION('center_axis',(0.,0.,1.));
#1970=DIRECTION('ref_axis',(1.,0.,0.));
#1971=DIRECTION('',(0.,0.,1.));
#1972=DIRECTION('center_axis',(0.,0.,1.));
#1973=DIRECTION('ref_axis',(1.,0.,0.));
#1974=DIRECTION('center_axis',(0.,0.,1.));
#1975=DIRECTION('ref_axis',(1.,0.,0.));
#1976=DIRECTION('',(0.,0.,1.));
#1977=DIRECTION('center_axis',(0.,0.,1.));
#1978=DIRECTION('ref_axis',(1.,0.,0.));
#1979=DIRECTION('center_axis',(0.,0.,1.));
#1980=DIRECTION('ref_axis',(1.,0.,0.));
#1981=DIRECTION('',(0.,0.,1.));
#1982=DIRECTION('center_axis',(0.,0.,1.));
#1983=DIRECTION('ref_axis',(1.,0.,0.));
#1984=DIRECTION('center_axis',(0.,0.,1.));
#1985=DIRECTION('ref_axis',(1.,0.,0.));
#1986=DIRECTION('',(0.,0.,1.));
#1987=DIRECTION('center_axis',(0.,0.,1.));
#1988=DIRECTION('ref_axis',(1.,0.,0.));
#1989=DIRECTION('center_axis',(0.,0.,1.));
#1990=DIRECTION('ref_axis',(1.,0.,0.));
#1991=DIRECTION('',(0.,0.,1.));
#1992=DIRECTION('center_axis',(0.,0.,1.));
#1993=DIRECTION('ref_axis',(1.,0.,0.));
#1994=DIRECTION('center_axis',(0.,0.,1.));
#1995=DIRECTION('ref_axis',(1.,0.,0.));
#1996=DIRECTION('',(0.,0.,1.));
#1997=DIRECTION('center_axis',(0.,0.,1.));
#1998=DIRECTION('ref_axis',(1.,0.,0.));
#1999=DIRECTION('center_axis',(0.,0.,1.));
#2000=DIRECTION('ref_axis',(1.,0.,0.));
#2001=DIRECTION('',(0.,0.,1.));
#2002=DIRECTION('center_axis',(0.,0.,1.));
#2003=DIRECTION('ref_axis',(1.,0.,0.));
#2004=DIRECTION('center_axis',(0.,0.,1.));
#2005=DIRECTION('ref_axis',(1.,0.,0.));
#2006=DIRECTION('',(0.,0.,1.));
#2007=DIRECTION('center_axis',(0.,0.,1.));
#2008=DIRECTION('ref_axis',(1.,0.,0.));
#2009=DIRECTION('center_axis',(0.,0.,1.));
#2010=DIRECTION('ref_axis',(1.,0.,0.));
#2011=DIRECTION('',(0.,0.,1.));
#2012=DIRECTION('center_axis',(0.,0.,1.));
#2013=DIRECTION('ref_axis',(1.,0.,0.));
#2014=DIRECTION('center_axis',(0.,0.,1.));
#2015=DIRECTION('ref_axis',(1.,0.,0.));
#2016=DIRECTION('',(0.,0.,1.));
#2017=DIRECTION('center_axis',(0.,0.,1.));
#2018=DIRECTION('ref_axis',(1.,0.,0.));
#2019=DIRECTION('center_axis',(0.,0.,1.));
#2020=DIRECTION('ref_axis',(1.,0.,0.));
#2021=DIRECTION('',(0.,0.,1.));
#2022=DIRECTION('center_axis',(0.,0.,1.));
#2023=DIRECTION('ref_axis',(1.,0.,0.));
#2024=DIRECTION('center_axis',(0.,0.,1.));
#2025=DIRECTION('ref_axis',(1.,0.,0.));
#2026=DIRECTION('',(0.,0.,1.));
#2027=DIRECTION('center_axis',(0.,0.,1.));
#2028=DIRECTION('ref_axis',(1.,0.,0.));
#2029=DIRECTION('center_axis',(0.,0.,1.));
#2030=DIRECTION('ref_axis',(1.,0.,0.));
#2031=DIRECTION('',(0.,0.,1.));
#2032=DIRECTION('center_axis',(0.,1.,0.));
#2033=DIRECTION('ref_axis',(-1.,0.,0.));
#2034=DIRECTION('',(-1.,0.,0.));
#2035=DIRECTION('',(0.,0.,1.));
#2036=DIRECTION('center_axis',(1.,0.,0.));
#2037=DIRECTION('ref_axis',(0.,1.,0.));
#2038=DIRECTION('',(0.,0.,1.));
#2039=DIRECTION('',(0.,1.,0.));
#2040=DIRECTION('center_axis',(0.,-1.,0.));
#2041=DIRECTION('ref_axis',(1.,0.,0.));
#2042=DIRECTION('',(1.,0.,0.));
#2043=DIRECTION('center_axis',(0.,0.,1.));
#2044=DIRECTION('ref_axis',(1.,0.,0.));
#2287=CARTESIAN_POINT('',(0.,0.,0.));
#2288=CARTESIAN_POINT('Origin',(-7.6,-0.5,1.5));
#2289=CARTESIAN_POINT('',(7.5,-0.5,0.9));
#2290=CARTESIAN_POINT('',(7.5,-0.5,1.4));
#2291=CARTESIAN_POINT('',(7.5,-0.5,0.75));
#2292=CARTESIAN_POINT('',(-7.5,-0.5,0.9));
#2293=CARTESIAN_POINT('',(-7.6,-0.5,0.9));
#2294=CARTESIAN_POINT('',(-7.5,-0.5,1.4));
#2295=CARTESIAN_POINT('',(-7.5,-0.5,0.75));
#2296=CARTESIAN_POINT('',(-3.8,-0.5,1.4));
#2297=CARTESIAN_POINT('Origin',(-7.6,-0.5,0.9));
#2298=CARTESIAN_POINT('',(7.5,-0.9,0.9));
#2299=CARTESIAN_POINT('',(7.5,-4.,0.9));
#2300=CARTESIAN_POINT('',(-7.5,-0.9,0.9));
#2301=CARTESIAN_POINT('',(-7.6,-0.9,0.9));
#2302=CARTESIAN_POINT('',(-7.5,3.5,0.9));
#2303=CARTESIAN_POINT('Origin',(-7.6,0.5,0.9));
#2304=CARTESIAN_POINT('',(7.5,0.5,1.4));
#2305=CARTESIAN_POINT('',(7.5,0.5,0.9));
#2306=CARTESIAN_POINT('',(7.5,0.5,0.45));
#2307=CARTESIAN_POINT('',(-7.5,0.5,1.4));
#2308=CARTESIAN_POINT('',(-3.8,0.5,1.4));
#2309=CARTESIAN_POINT('',(-7.5,0.5,0.9));
#2310=CARTESIAN_POINT('',(-7.5,0.5,0.45));
#2311=CARTESIAN_POINT('',(-7.6,0.5,0.9));
#2312=CARTESIAN_POINT('Origin',(-7.6,0.9,0.9));
#2313=CARTESIAN_POINT('',(7.5,0.9,0.9));
#2314=CARTESIAN_POINT('',(7.5,-3.3,0.9));
#2315=CARTESIAN_POINT('',(-7.5,0.9,0.9));
#2316=CARTESIAN_POINT('',(-7.5,4.2,0.9));
#2317=CARTESIAN_POINT('',(-7.6,0.9,0.9));
#2318=CARTESIAN_POINT('Origin',(-7.6,0.9,0.3));
#2319=CARTESIAN_POINT('',(7.5,0.9,0.3));
#2320=CARTESIAN_POINT('',(7.5,0.9,0.15));
#2321=CARTESIAN_POINT('',(-7.5,0.9,0.3));
#2322=CARTESIAN_POINT('',(-7.5,0.9,0.15));
#2323=CARTESIAN_POINT('',(-7.6,0.9,0.3));
#2324=CARTESIAN_POINT('Origin',(-7.6,-0.9,0.3));
#2325=CARTESIAN_POINT('',(7.5,-0.9,0.3));
#2326=CARTESIAN_POINT('',(7.5,-4.2,0.3));
#2327=CARTESIAN_POINT('',(-7.5,-0.9,0.3));
#2328=CARTESIAN_POINT('',(-7.5,3.3,0.3));
#2329=CARTESIAN_POINT('',(-7.6,-0.9,0.3));
#2330=CARTESIAN_POINT('Origin',(-7.6,-0.9,0.9));
#2331=CARTESIAN_POINT('',(7.5,-0.9,0.45));
#2332=CARTESIAN_POINT('',(-7.5,-0.9,0.45));
#2333=CARTESIAN_POINT('Origin',(-7.5,7.5,0.));
#2334=CARTESIAN_POINT('',(-7.5,7.5,1.4));
#2335=CARTESIAN_POINT('',(-7.5,7.5,1.4));
#2336=CARTESIAN_POINT('',(-7.5,7.5,0.));
#2337=CARTESIAN_POINT('',(-7.5,7.5,0.));
#2338=CARTESIAN_POINT('',(-7.5,-7.5,0.));
#2339=CARTESIAN_POINT('',(-7.5,7.5,0.));
#2340=CARTESIAN_POINT('',(-7.5,-7.5,1.4));
#2341=CARTESIAN_POINT('',(-7.5,-7.5,0.));
#2342=CARTESIAN_POINT('',(-7.5,7.5,1.4));
#2343=CARTESIAN_POINT('Origin',(0.,0.,1.4));
#2344=CARTESIAN_POINT('',(7.5,7.5,1.4));
#2345=CARTESIAN_POINT('',(7.5,-7.5,1.4));
#2346=CARTESIAN_POINT('',(7.5,7.5,1.4));
#2347=CARTESIAN_POINT('',(4.66,2.5,1.4));
#2348=CARTESIAN_POINT('Origin',(5.,2.5,1.4));
#2349=CARTESIAN_POINT('',(2.16,2.5,1.4));
#2350=CARTESIAN_POINT('Origin',(2.5,2.5,1.4));
#2351=CARTESIAN_POINT('',(-0.34,2.5,1.4));
#2352=CARTESIAN_POINT('Origin',(0.,2.5,1.4));
#2353=CARTESIAN_POINT('',(-2.84,5.,1.4));
#2354=CARTESIAN_POINT('Origin',(-2.5,5.,1.4));
#2355=CARTESIAN_POINT('',(-5.34,5.,1.4));
#2356=CARTESIAN_POINT('Origin',(-5.,5.,1.4));
#2357=CARTESIAN_POINT('',(-5.34,2.5,1.4));
#2358=CARTESIAN_POINT('Origin',(-5.,2.5,1.4));
#2359=CARTESIAN_POINT('',(-2.84,2.5,1.4));
#2360=CARTESIAN_POINT('Origin',(-2.5,2.5,1.4));
#2361=CARTESIAN_POINT('',(-0.34,5.,1.4));
#2362=CARTESIAN_POINT('Origin',(0.,5.,1.4));
#2363=CARTESIAN_POINT('',(2.16,5.,1.4));
#2364=CARTESIAN_POINT('Origin',(2.5,5.,1.4));
#2365=CARTESIAN_POINT('',(4.66,5.,1.4));
#2366=CARTESIAN_POINT('Origin',(5.,5.,1.4));
#2367=CARTESIAN_POINT('Origin',(0.,0.,1.4));
#2368=CARTESIAN_POINT('',(7.5,-7.5,1.4));
#2369=CARTESIAN_POINT('',(-7.5,-7.5,1.4));
#2370=CARTESIAN_POINT('',(7.5,-7.5,1.4));
#2371=CARTESIAN_POINT('',(4.66,-5.,1.4));
#2372=CARTESIAN_POINT('Origin',(5.,-5.,1.4));
#2373=CARTESIAN_POINT('',(2.16,-5.,1.4));
#2374=CARTESIAN_POINT('Origin',(2.5,-5.,1.4));
#2375=CARTESIAN_POINT('',(-0.34,-2.5,1.4));
#2376=CARTESIAN_POINT('Origin',(0.,-2.5,1.4));
#2377=CARTESIAN_POINT('',(-2.84,-2.5,1.4));
#2378=CARTESIAN_POINT('Origin',(-2.5,-2.5,1.4));
#2379=CARTESIAN_POINT('',(-5.34,-2.5,1.4));
#2380=CARTESIAN_POINT('Origin',(-5.,-2.5,1.4));
#2381=CARTESIAN_POINT('',(-2.84,-5.,1.4));
#2382=CARTESIAN_POINT('Origin',(-2.5,-5.,1.4));
#2383=CARTESIAN_POINT('',(-0.34,-5.,1.4));
#2384=CARTESIAN_POINT('Origin',(0.,-5.,1.4));
#2385=CARTESIAN_POINT('',(-5.34,-5.,1.4));
#2386=CARTESIAN_POINT('Origin',(-5.,-5.,1.4));
#2387=CARTESIAN_POINT('',(2.16,-2.5,1.4));
#2388=CARTESIAN_POINT('Origin',(2.5,-2.5,1.4));
#2389=CARTESIAN_POINT('',(4.66,-2.5,1.4));
#2390=CARTESIAN_POINT('Origin',(5.,-2.5,1.4));
#2391=CARTESIAN_POINT('Origin',(5.,2.5,-0.1));
#2392=CARTESIAN_POINT('',(4.66,2.5,0.));
#2393=CARTESIAN_POINT('Origin',(5.,2.5,0.));
#2394=CARTESIAN_POINT('',(4.66,2.5,-0.1));
#2395=CARTESIAN_POINT('Origin',(5.,-5.,-0.1));
#2396=CARTESIAN_POINT('',(4.66,-5.,0.));
#2397=CARTESIAN_POINT('Origin',(5.,-5.,0.));
#2398=CARTESIAN_POINT('',(4.66,-5.,-0.1));
#2399=CARTESIAN_POINT('Origin',(2.5,2.5,-0.1));
#2400=CARTESIAN_POINT('',(2.16,2.5,0.));
#2401=CARTESIAN_POINT('Origin',(2.5,2.5,0.));
#2402=CARTESIAN_POINT('',(2.16,2.5,-0.1));
#2403=CARTESIAN_POINT('Origin',(2.5,-5.,-0.1));
#2404=CARTESIAN_POINT('',(2.16,-5.,0.));
#2405=CARTESIAN_POINT('Origin',(2.5,-5.,0.));
#2406=CARTESIAN_POINT('',(2.16,-5.,-0.1));
#2407=CARTESIAN_POINT('Origin',(0.,2.5,-0.1));
#2408=CARTESIAN_POINT('',(-0.34,2.5,0.));
#2409=CARTESIAN_POINT('Origin',(0.,2.5,0.));
#2410=CARTESIAN_POINT('',(-0.34,2.5,-0.1));
#2411=CARTESIAN_POINT('Origin',(0.,-2.5,-0.1));
#2412=CARTESIAN_POINT('',(-0.34,-2.5,0.));
#2413=CARTESIAN_POINT('Origin',(0.,-2.5,0.));
#2414=CARTESIAN_POINT('',(-0.34,-2.5,-0.1));
#2415=CARTESIAN_POINT('Origin',(-2.5,5.,-0.1));
#2416=CARTESIAN_POINT('',(-2.84,5.,0.));
#2417=CARTESIAN_POINT('Origin',(-2.5,5.,0.));
#2418=CARTESIAN_POINT('',(-2.84,5.,-0.1));
#2419=CARTESIAN_POINT('Origin',(-2.5,-2.5,-0.1));
#2420=CARTESIAN_POINT('',(-2.84,-2.5,0.));
#2421=CARTESIAN_POINT('Origin',(-2.5,-2.5,0.));
#2422=CARTESIAN_POINT('',(-2.84,-2.5,-0.1));
#2423=CARTESIAN_POINT('Origin',(-5.,5.,-0.1));
#2424=CARTESIAN_POINT('',(-5.34,5.,0.));
#2425=CARTESIAN_POINT('Origin',(-5.,5.,0.));
#2426=CARTESIAN_POINT('',(-5.34,5.,-0.1));
#2427=CARTESIAN_POINT('Origin',(-5.,-2.5,-0.1));
#2428=CARTESIAN_POINT('',(-5.34,-2.5,0.));
#2429=CARTESIAN_POINT('Origin',(-5.,-2.5,0.));
#2430=CARTESIAN_POINT('',(-5.34,-2.5,-0.1));
#2431=CARTESIAN_POINT('Origin',(-5.,2.5,-0.1));
#2432=CARTESIAN_POINT('',(-5.34,2.5,0.));
#2433=CARTESIAN_POINT('Origin',(-5.,2.5,0.));
#2434=CARTESIAN_POINT('',(-5.34,2.5,-0.1));
#2435=CARTESIAN_POINT('Origin',(-2.5,-5.,-0.1));
#2436=CARTESIAN_POINT('',(-2.84,-5.,0.));
#2437=CARTESIAN_POINT('Origin',(-2.5,-5.,0.));
#2438=CARTESIAN_POINT('',(-2.84,-5.,-0.1));
#2439=CARTESIAN_POINT('Origin',(-2.5,2.5,-0.1));
#2440=CARTESIAN_POINT('',(-2.84,2.5,0.));
#2441=CARTESIAN_POINT('Origin',(-2.5,2.5,0.));
#2442=CARTESIAN_POINT('',(-2.84,2.5,-0.1));
#2443=CARTESIAN_POINT('Origin',(0.,-5.,-0.1));
#2444=CARTESIAN_POINT('',(-0.34,-5.,0.));
#2445=CARTESIAN_POINT('Origin',(0.,-5.,0.));
#2446=CARTESIAN_POINT('',(-0.34,-5.,-0.1));
#2447=CARTESIAN_POINT('Origin',(-5.,-5.,-0.1));
#2448=CARTESIAN_POINT('',(-5.34,-5.,0.));
#2449=CARTESIAN_POINT('Origin',(-5.,-5.,0.));
#2450=CARTESIAN_POINT('',(-5.34,-5.,-0.1));
#2451=CARTESIAN_POINT('Origin',(0.,5.,-0.1));
#2452=CARTESIAN_POINT('',(-0.34,5.,0.));
#2453=CARTESIAN_POINT('Origin',(0.,5.,0.));
#2454=CARTESIAN_POINT('',(-0.34,5.,-0.1));
#2455=CARTESIAN_POINT('Origin',(2.5,-2.5,-0.1));
#2456=CARTESIAN_POINT('',(2.16,-2.5,0.));
#2457=CARTESIAN_POINT('Origin',(2.5,-2.5,0.));
#2458=CARTESIAN_POINT('',(2.16,-2.5,-0.1));
#2459=CARTESIAN_POINT('Origin',(2.5,5.,-0.1));
#2460=CARTESIAN_POINT('',(2.16,5.,0.));
#2461=CARTESIAN_POINT('Origin',(2.5,5.,0.));
#2462=CARTESIAN_POINT('',(2.16,5.,-0.1));
#2463=CARTESIAN_POINT('Origin',(5.,-2.5,-0.1));
#2464=CARTESIAN_POINT('',(4.66,-2.5,0.));
#2465=CARTESIAN_POINT('Origin',(5.,-2.5,0.));
#2466=CARTESIAN_POINT('',(4.66,-2.5,-0.1));
#2467=CARTESIAN_POINT('Origin',(5.,5.,-0.1));
#2468=CARTESIAN_POINT('',(4.66,5.,0.));
#2469=CARTESIAN_POINT('Origin',(5.,5.,0.));
#2470=CARTESIAN_POINT('',(4.66,5.,-0.1));
#2471=CARTESIAN_POINT('Origin',(7.5,7.5,0.));
#2472=CARTESIAN_POINT('',(7.5,7.5,0.));
#2473=CARTESIAN_POINT('',(7.5,7.5,0.));
#2474=CARTESIAN_POINT('',(7.5,7.5,0.));
#2475=CARTESIAN_POINT('Origin',(7.5,-7.5,0.));
#2476=CARTESIAN_POINT('',(7.5,-7.5,0.));
#2477=CARTESIAN_POINT('',(7.5,-7.5,0.));
#2478=CARTESIAN_POINT('',(7.5,-7.5,0.));
#2479=CARTESIAN_POINT('Origin',(-7.5,-7.5,0.));
#2480=CARTESIAN_POINT('',(-7.5,-7.5,0.));
#2481=CARTESIAN_POINT('Origin',(0.,0.,0.));
#2752=UNCERTAINTY_MEASURE_WITH_UNIT(LENGTH_MEASURE(0.001),#2769,
'DISTANCE_ACCURACY_VALUE',
'Maximum model space distance between geometric entities at asserted c
onnectivities');
#2759=UNCERTAINTY_MEASURE_WITH_UNIT(LENGTH_MEASURE(0.001),#2769,
'DISTANCE_ACCURACY_VALUE',
'Maximum model space distance between geometric entities at asserted c
onnectivities');
#2761=(
GEOMETRIC_REPRESENTATION_CONTEXT(3)
GLOBAL_UNCERTAINTY_ASSIGNED_CONTEXT((#2752))
GLOBAL_UNIT_ASSIGNED_CONTEXT((#2769,#2771,#2772))
REPRESENTATION_CONTEXT('','3D')
);
#2768=(
GEOMETRIC_REPRESENTATION_CONTEXT(3)
GLOBAL_UNCERTAINTY_ASSIGNED_CONTEXT((#2759))
GLOBAL_UNIT_ASSIGNED_CONTEXT((#2769,#2771,#2772))
REPRESENTATION_CONTEXT('','3D')
);
#2769=(
LENGTH_UNIT()
NAMED_UNIT(*)
SI_UNIT(.CENTI.,.METRE.)
);
#2771=(
NAMED_UNIT(*)
PLANE_ANGLE_UNIT()
SI_UNIT($,.RADIAN.)
);
#2772=(
NAMED_UNIT(*)
SI_UNIT($,.STERADIAN.)
SOLID_ANGLE_UNIT()
);
#2774=SHAPE_DEFINITION_REPRESENTATION(#2782,#2799);
#2782=PRODUCT_DEFINITION_SHAPE('',$,#2808);
#2799=SHAPE_REPRESENTATION('',(#1682),#2761);
#2806=PRODUCT_DEFINITION_CONTEXT('part definition',#2832,'design');
#2808=PRODUCT_DEFINITION('Slotted grid plate','Slotted grid plate',
#2816,#2806);
#2816=PRODUCT_DEFINITION_FORMATION('',$,#2835);
#2832=APPLICATION_CONTEXT(
'Core Data for Automotive Mechanical Design Process');
#2833=PRODUCT_CONTEXT('part definition',#2832,'mechanical');
#2835=PRODUCT('Slotted grid plate','Slotted grid plate',
'Slotted grid plate',(#2833));
#2919=COLOUR_RGB('Off White',0.89,0.88,0.83);
#2920=FILL_AREA_STYLE_COLOUR('',#2919);
#2921=FILL_AREA_STYLE('',(#2920));
#2922=SURFACE_STYLE_FILL_AREA(#2921);
#2923=SURFACE_SIDE_STYLE('',(#2922));
#2924=SURFACE_STYLE_USAGE(.BOTH.,#2923);
#2925=PRESENTATION_STYLE_ASSIGNMENT((#2924));
ENDSEC;
END-ISO-10303-21;
